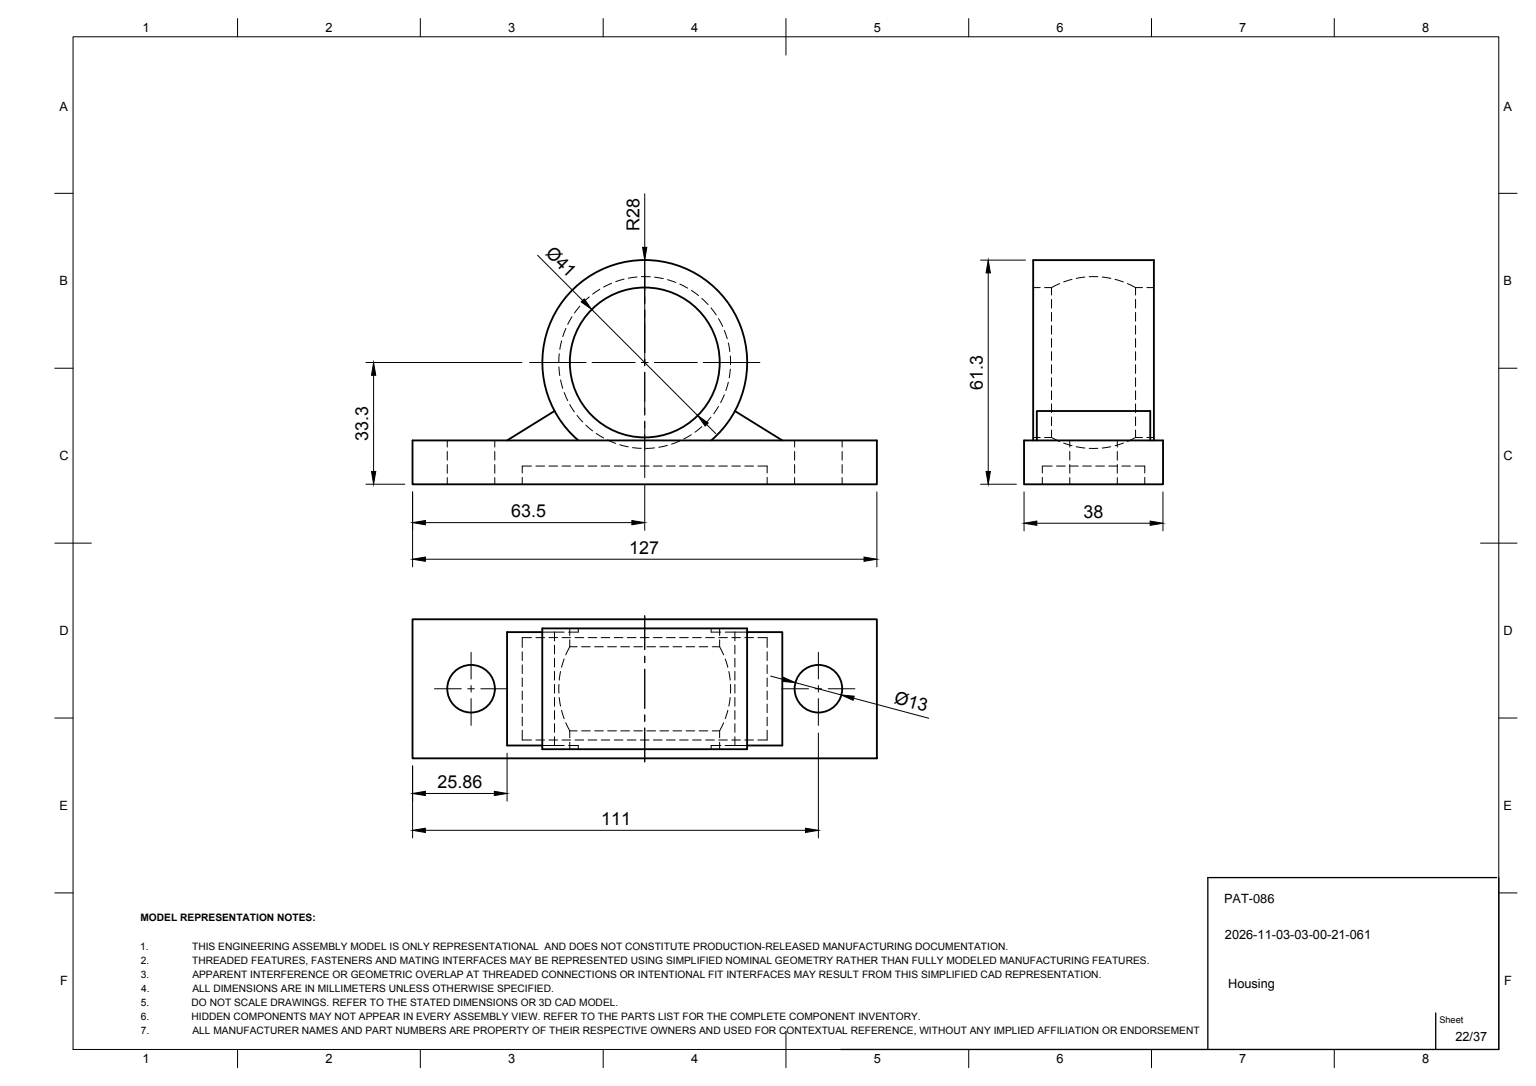
ISO-10303-21;
HEADER;
/* Generated by software containing ST-Developer
 * from STEP Tools, Inc. (www.steptools.com) 
 */

FILE_DESCRIPTION(
/* description */ ('Ratchet and pawl hand winch drum'),
/* implementation_level */ '2;1');

FILE_NAME(
/* name */ 'Housing.step',
/* time_stamp */ '2026-10-27T12:42:58-07:00',
/* author */ (''),
/* organization */ (''),
/* preprocessor_version */ 'ST-DEVELOPER v20.2',
/* originating_system */ 'Autodesk Translation Framework v15.17.0.0',
/* authorisation */ '');

FILE_SCHEMA (('AUTOMOTIVE_DESIGN { 1 0 10303 214 3 1 1 }'));
ENDSEC;

DATA;
#10=MECHANICAL_DESIGN_GEOMETRIC_PRESENTATION_REPRESENTATION('',(#404),#11801);
#319=SPHERICAL_SURFACE('',#6928,2.35);
#336=SHAPE_REPRESENTATION_RELATIONSHIP('SRR','None',#11963,#370);
#370=ADVANCED_BREP_SHAPE_REPRESENTATION('',(#439),#11780);
#404=STYLED_ITEM('',(#12192),#439);
#439=MANIFOLD_SOLID_BREP('Body1',#6281);
#531=FACE_BOUND('',#1400,.T.);
#532=FACE_BOUND('',#1401,.T.);
#533=FACE_BOUND('',#1409,.T.);
#534=FACE_BOUND('',#1410,.T.);
#535=FACE_BOUND('',#1411,.T.);
#536=FACE_BOUND('',#1414,.T.);
#537=FACE_BOUND('',#1416,.T.);
#538=FACE_BOUND('',#1429,.T.);
#539=FACE_BOUND('',#1430,.T.);
#540=FACE_BOUND('',#1431,.T.);
#678=PLANE('',#6930);
#679=PLANE('',#6932);
#680=PLANE('',#6934);
#681=PLANE('',#6936);
#682=PLANE('',#6937);
#683=PLANE('',#6939);
#684=PLANE('',#6940);
#685=PLANE('',#6946);
#686=PLANE('',#6947);
#687=PLANE('',#6948);
#688=PLANE('',#6949);
#689=PLANE('',#6950);
#690=PLANE('',#6951);
#691=PLANE('',#6952);
#692=PLANE('',#6957);
#693=PLANE('',#6958);
#694=PLANE('',#6959);
#695=PLANE('',#6960);
#696=PLANE('',#6961);
#966=FACE_OUTER_BOUND('',#1397,.T.);
#967=FACE_OUTER_BOUND('',#1398,.T.);
#968=FACE_OUTER_BOUND('',#1399,.T.);
#969=FACE_OUTER_BOUND('',#1402,.T.);
#970=FACE_OUTER_BOUND('',#1403,.T.);
#971=FACE_OUTER_BOUND('',#1404,.T.);
#972=FACE_OUTER_BOUND('',#1405,.T.);
#973=FACE_OUTER_BOUND('',#1406,.T.);
#974=FACE_OUTER_BOUND('',#1407,.T.);
#975=FACE_OUTER_BOUND('',#1408,.T.);
#976=FACE_OUTER_BOUND('',#1412,.T.);
#977=FACE_OUTER_BOUND('',#1413,.T.);
#978=FACE_OUTER_BOUND('',#1415,.T.);
#979=FACE_OUTER_BOUND('',#1417,.T.);
#980=FACE_OUTER_BOUND('',#1418,.T.);
#981=FACE_OUTER_BOUND('',#1419,.T.);
#982=FACE_OUTER_BOUND('',#1420,.T.);
#983=FACE_OUTER_BOUND('',#1421,.T.);
#984=FACE_OUTER_BOUND('',#1422,.T.);
#985=FACE_OUTER_BOUND('',#1423,.T.);
#986=FACE_OUTER_BOUND('',#1424,.T.);
#987=FACE_OUTER_BOUND('',#1425,.T.);
#988=FACE_OUTER_BOUND('',#1426,.T.);
#989=FACE_OUTER_BOUND('',#1427,.T.);
#990=FACE_OUTER_BOUND('',#1428,.T.);
#1397=EDGE_LOOP('',(#4757,#4758,#4759,#4760));
#1398=EDGE_LOOP('',(#4761,#4762,#4763,#4764));
#1399=EDGE_LOOP('',(#4765,#4766));
#1400=EDGE_LOOP('',(#4767));
#1401=EDGE_LOOP('',(#4768));
#1402=EDGE_LOOP('',(#4769,#4770,#4771));
#1403=EDGE_LOOP('',(#4772,#4773,#4774));
#1404=EDGE_LOOP('',(#4775,#4776,#4777));
#1405=EDGE_LOOP('',(#4778,#4779,#4780,#4781));
#1406=EDGE_LOOP('',(#4782,#4783,#4784));
#1407=EDGE_LOOP('',(#4785,#4786,#4787,#4788));
#1408=EDGE_LOOP('',(#4789,#4790,#4791,#4792));
#1409=EDGE_LOOP('',(#4793));
#1410=EDGE_LOOP('',(#4794));
#1411=EDGE_LOOP('',(#4795,#4796,#4797,#4798,#4799,#4800,#4801,#4802,#4803,
#4804,#4805,#4806));
#1412=EDGE_LOOP('',(#4807,#4808,#4809,#4810,#4811,#4812,#4813,#4814,#4815,
#4816,#4817,#4818));
#1413=EDGE_LOOP('',(#4819,#4820));
#1414=EDGE_LOOP('',(#4821));
#1415=EDGE_LOOP('',(#4822,#4823));
#1416=EDGE_LOOP('',(#4824));
#1417=EDGE_LOOP('',(#4825,#4826,#4827,#4828));
#1418=EDGE_LOOP('',(#4829,#4830,#4831,#4832));
#1419=EDGE_LOOP('',(#4833,#4834,#4835,#4836));
#1420=EDGE_LOOP('',(#4837,#4838,#4839,#4840));
#1421=EDGE_LOOP('',(#4841,#4842,#4843,#4844));
#1422=EDGE_LOOP('',(#4845,#4846,#4847,#4848));
#1423=EDGE_LOOP('',(#4849,#4850,#4851,#4852));
#1424=EDGE_LOOP('',(#4853,#4854,#4855,#4856));
#1425=EDGE_LOOP('',(#4857,#4858,#4859,#4860));
#1426=EDGE_LOOP('',(#4861,#4862,#4863,#4864));
#1427=EDGE_LOOP('',(#4865,#4866,#4867,#4868));
#1428=EDGE_LOOP('',(#4869,#4870,#4871,#4872));
#1429=EDGE_LOOP('',(#4873,#4874,#4875,#4876));
#1430=EDGE_LOOP('',(#4877));
#1431=EDGE_LOOP('',(#4878));
#1854=LINE('',#9801,#2365);
#1855=LINE('',#9807,#2366);
#1856=LINE('',#9816,#2367);
#1857=LINE('',#9818,#2368);
#1858=LINE('',#9823,#2369);
#1859=LINE('',#9826,#2370);
#1860=LINE('',#9830,#2371);
#1861=LINE('',#9833,#2372);
#1862=LINE('',#9835,#2373);
#1863=LINE('',#9836,#2374);
#1864=LINE('',#9840,#2375);
#1865=LINE('',#9842,#2376);
#1866=LINE('',#9845,#2377);
#1867=LINE('',#9846,#2378);
#1868=LINE('',#9850,#2379);
#1869=LINE('',#9852,#2380);
#1870=LINE('',#9854,#2381);
#1871=LINE('',#9855,#2382);
#1872=LINE('',#9861,#2383);
#1873=LINE('',#9863,#2384);
#1874=LINE('',#9864,#2385);
#1875=LINE('',#9866,#2386);
#1876=LINE('',#9868,#2387);
#1877=LINE('',#9869,#2388);
#1878=LINE('',#9878,#2389);
#1879=LINE('',#9880,#2390);
#1880=LINE('',#9882,#2391);
#1881=LINE('',#9883,#2392);
#1882=LINE('',#9886,#2393);
#1883=LINE('',#9888,#2394);
#1884=LINE('',#9889,#2395);
#1885=LINE('',#9892,#2396);
#1886=LINE('',#9894,#2397);
#1887=LINE('',#9895,#2398);
#1888=LINE('',#9897,#2399);
#1889=LINE('',#9898,#2400);
#1890=LINE('',#9903,#2401);
#1891=LINE('',#9907,#2402);
#1892=LINE('',#9911,#2403);
#1893=LINE('',#9912,#2404);
#1894=LINE('',#9913,#2405);
#1895=LINE('',#9916,#2406);
#1896=LINE('',#9917,#2407);
#1897=LINE('',#9920,#2408);
#1898=LINE('',#9921,#2409);
#1899=LINE('',#9923,#2410);
#2365=VECTOR('',#8005,2.05);
#2366=VECTOR('',#8012,2.05);
#2367=VECTOR('',#8021,1.);
#2368=VECTOR('',#8022,1.);
#2369=VECTOR('',#8027,1.);
#2370=VECTOR('',#8030,1.);
#2371=VECTOR('',#8033,1.);
#2372=VECTOR('',#8036,1.);
#2373=VECTOR('',#8039,1.);
#2374=VECTOR('',#8040,1.);
#2375=VECTOR('',#8043,1.);
#2376=VECTOR('',#8044,1.);
#2377=VECTOR('',#8049,1.);
#2378=VECTOR('',#8050,1.);
#2379=VECTOR('',#8053,1.);
#2380=VECTOR('',#8054,1.);
#2381=VECTOR('',#8055,1.);
#2382=VECTOR('',#8056,1.);
#2383=VECTOR('',#8061,1.);
#2384=VECTOR('',#8062,1.);
#2385=VECTOR('',#8063,1.);
#2386=VECTOR('',#8064,1.);
#2387=VECTOR('',#8065,1.);
#2388=VECTOR('',#8066,1.);
#2389=VECTOR('',#8079,1.);
#2390=VECTOR('',#8080,1.);
#2391=VECTOR('',#8081,1.);
#2392=VECTOR('',#8082,1.);
#2393=VECTOR('',#8085,1.);
#2394=VECTOR('',#8086,1.);
#2395=VECTOR('',#8087,1.);
#2396=VECTOR('',#8090,1.);
#2397=VECTOR('',#8091,1.);
#2398=VECTOR('',#8092,1.);
#2399=VECTOR('',#8095,1.);
#2400=VECTOR('',#8096,1.);
#2401=VECTOR('',#8103,0.65);
#2402=VECTOR('',#8108,0.65);
#2403=VECTOR('',#8111,1.);
#2404=VECTOR('',#8112,1.);
#2405=VECTOR('',#8113,1.);
#2406=VECTOR('',#8116,1.);
#2407=VECTOR('',#8117,1.);
#2408=VECTOR('',#8120,1.);
#2409=VECTOR('',#8121,1.);
#2410=VECTOR('',#8124,1.);
#2817=CIRCLE('',#6923,2.05);
#2818=CIRCLE('',#6924,2.05);
#2819=CIRCLE('',#6926,2.05);
#2820=CIRCLE('',#6927,2.05);
#2821=CIRCLE('',#6929,2.35);
#2822=CIRCLE('',#6931,2.8);
#2823=CIRCLE('',#6933,2.8);
#2824=CIRCLE('',#6935,2.8);
#2825=CIRCLE('',#6938,2.8);
#2826=CIRCLE('',#6941,0.65);
#2827=CIRCLE('',#6942,0.65);
#2828=CIRCLE('',#6944,2.8);
#2829=CIRCLE('',#6945,2.8);
#2830=CIRCLE('',#6954,0.65);
#2831=CIRCLE('',#6956,0.65);
#3112=VERTEX_POINT('',#9798);
#3113=VERTEX_POINT('',#9800);
#3114=VERTEX_POINT('',#9804);
#3115=VERTEX_POINT('',#9806);
#3116=VERTEX_POINT('',#9810);
#3117=VERTEX_POINT('',#9811);
#3118=VERTEX_POINT('',#9814);
#3119=VERTEX_POINT('',#9815);
#3120=VERTEX_POINT('',#9817);
#3121=VERTEX_POINT('',#9821);
#3122=VERTEX_POINT('',#9822);
#3123=VERTEX_POINT('',#9824);
#3124=VERTEX_POINT('',#9828);
#3125=VERTEX_POINT('',#9829);
#3126=VERTEX_POINT('',#9831);
#3127=VERTEX_POINT('',#9838);
#3128=VERTEX_POINT('',#9839);
#3129=VERTEX_POINT('',#9841);
#3130=VERTEX_POINT('',#9848);
#3131=VERTEX_POINT('',#9849);
#3132=VERTEX_POINT('',#9851);
#3133=VERTEX_POINT('',#9853);
#3134=VERTEX_POINT('',#9856);
#3135=VERTEX_POINT('',#9858);
#3136=VERTEX_POINT('',#9860);
#3137=VERTEX_POINT('',#9862);
#3138=VERTEX_POINT('',#9865);
#3139=VERTEX_POINT('',#9867);
#3140=VERTEX_POINT('',#9876);
#3141=VERTEX_POINT('',#9877);
#3142=VERTEX_POINT('',#9879);
#3143=VERTEX_POINT('',#9881);
#3144=VERTEX_POINT('',#9885);
#3145=VERTEX_POINT('',#9887);
#3146=VERTEX_POINT('',#9891);
#3147=VERTEX_POINT('',#9893);
#3148=VERTEX_POINT('',#9901);
#3149=VERTEX_POINT('',#9905);
#3150=VERTEX_POINT('',#9909);
#3151=VERTEX_POINT('',#9910);
#3152=VERTEX_POINT('',#9915);
#3153=VERTEX_POINT('',#9919);
#3722=EDGE_CURVE('',#3112,#3112,#2817,.T.);
#3723=EDGE_CURVE('',#3112,#3113,#1854,.T.);
#3724=EDGE_CURVE('',#3113,#3113,#2818,.T.);
#3725=EDGE_CURVE('',#3114,#3114,#2819,.T.);
#3726=EDGE_CURVE('',#3114,#3115,#1855,.T.);
#3727=EDGE_CURVE('',#3115,#3115,#2820,.T.);
#3728=EDGE_CURVE('',#3116,#3117,#2821,.T.);
#3729=EDGE_CURVE('',#3118,#3119,#1856,.T.);
#3730=EDGE_CURVE('',#3118,#3120,#1857,.T.);
#3731=EDGE_CURVE('',#3119,#3120,#2822,.T.);
#3732=EDGE_CURVE('',#3121,#3122,#1858,.T.);
#3733=EDGE_CURVE('',#3123,#3121,#2823,.T.);
#3734=EDGE_CURVE('',#3123,#3122,#1859,.T.);
#3735=EDGE_CURVE('',#3124,#3125,#1860,.T.);
#3736=EDGE_CURVE('',#3126,#3124,#2824,.T.);
#3737=EDGE_CURVE('',#3126,#3125,#1861,.T.);
#3738=EDGE_CURVE('',#3125,#3118,#1862,.T.);
#3739=EDGE_CURVE('',#3120,#3126,#1863,.T.);
#3740=EDGE_CURVE('',#3127,#3128,#1864,.T.);
#3741=EDGE_CURVE('',#3127,#3129,#1865,.T.);
#3742=EDGE_CURVE('',#3128,#3129,#2825,.T.);
#3743=EDGE_CURVE('',#3122,#3127,#1866,.T.);
#3744=EDGE_CURVE('',#3129,#3123,#1867,.T.);
#3745=EDGE_CURVE('',#3130,#3131,#1868,.T.);
#3746=EDGE_CURVE('',#3131,#3132,#1869,.T.);
#3747=EDGE_CURVE('',#3132,#3133,#1870,.T.);
#3748=EDGE_CURVE('',#3133,#3130,#1871,.T.);
#3749=EDGE_CURVE('',#3134,#3134,#2826,.T.);
#3750=EDGE_CURVE('',#3135,#3135,#2827,.T.);
#3751=EDGE_CURVE('',#3128,#3136,#1872,.T.);
#3752=EDGE_CURVE('',#3136,#3137,#1873,.T.);
#3753=EDGE_CURVE('',#3137,#3124,#1874,.T.);
#3754=EDGE_CURVE('',#3119,#3138,#1875,.T.);
#3755=EDGE_CURVE('',#3138,#3139,#1876,.T.);
#3756=EDGE_CURVE('',#3139,#3121,#1877,.T.);
#3757=EDGE_CURVE('',#3138,#3139,#2828,.T.);
#3758=EDGE_CURVE('',#3136,#3137,#2829,.T.);
#3759=EDGE_CURVE('',#3140,#3141,#1878,.T.);
#3760=EDGE_CURVE('',#3140,#3142,#1879,.T.);
#3761=EDGE_CURVE('',#3142,#3143,#1880,.T.);
#3762=EDGE_CURVE('',#3141,#3143,#1881,.T.);
#3763=EDGE_CURVE('',#3144,#3140,#1882,.T.);
#3764=EDGE_CURVE('',#3144,#3145,#1883,.T.);
#3765=EDGE_CURVE('',#3145,#3142,#1884,.T.);
#3766=EDGE_CURVE('',#3146,#3144,#1885,.T.);
#3767=EDGE_CURVE('',#3146,#3147,#1886,.T.);
#3768=EDGE_CURVE('',#3147,#3145,#1887,.T.);
#3769=EDGE_CURVE('',#3141,#3146,#1888,.T.);
#3770=EDGE_CURVE('',#3143,#3147,#1889,.T.);
#3771=EDGE_CURVE('',#3148,#3148,#2830,.T.);
#3772=EDGE_CURVE('',#3148,#3135,#1890,.T.);
#3773=EDGE_CURVE('',#3149,#3149,#2831,.T.);
#3774=EDGE_CURVE('',#3149,#3134,#1891,.T.);
#3775=EDGE_CURVE('',#3150,#3151,#1892,.T.);
#3776=EDGE_CURVE('',#3151,#3130,#1893,.T.);
#3777=EDGE_CURVE('',#3150,#3133,#1894,.T.);
#3778=EDGE_CURVE('',#3152,#3150,#1895,.T.);
#3779=EDGE_CURVE('',#3152,#3132,#1896,.T.);
#3780=EDGE_CURVE('',#3153,#3152,#1897,.T.);
#3781=EDGE_CURVE('',#3153,#3131,#1898,.T.);
#3782=EDGE_CURVE('',#3151,#3153,#1899,.T.);
#4757=ORIENTED_EDGE('',*,*,#3722,.F.);
#4758=ORIENTED_EDGE('',*,*,#3723,.T.);
#4759=ORIENTED_EDGE('',*,*,#3724,.F.);
#4760=ORIENTED_EDGE('',*,*,#3723,.F.);
#4761=ORIENTED_EDGE('',*,*,#3725,.F.);
#4762=ORIENTED_EDGE('',*,*,#3726,.T.);
#4763=ORIENTED_EDGE('',*,*,#3727,.F.);
#4764=ORIENTED_EDGE('',*,*,#3726,.F.);
#4765=ORIENTED_EDGE('',*,*,#3728,.T.);
#4766=ORIENTED_EDGE('',*,*,#3728,.F.);
#4767=ORIENTED_EDGE('',*,*,#3725,.T.);
#4768=ORIENTED_EDGE('',*,*,#3724,.T.);
#4769=ORIENTED_EDGE('',*,*,#3729,.F.);
#4770=ORIENTED_EDGE('',*,*,#3730,.T.);
#4771=ORIENTED_EDGE('',*,*,#3731,.F.);
#4772=ORIENTED_EDGE('',*,*,#3732,.F.);
#4773=ORIENTED_EDGE('',*,*,#3733,.F.);
#4774=ORIENTED_EDGE('',*,*,#3734,.T.);
#4775=ORIENTED_EDGE('',*,*,#3735,.F.);
#4776=ORIENTED_EDGE('',*,*,#3736,.F.);
#4777=ORIENTED_EDGE('',*,*,#3737,.T.);
#4778=ORIENTED_EDGE('',*,*,#3738,.F.);
#4779=ORIENTED_EDGE('',*,*,#3737,.F.);
#4780=ORIENTED_EDGE('',*,*,#3739,.F.);
#4781=ORIENTED_EDGE('',*,*,#3730,.F.);
#4782=ORIENTED_EDGE('',*,*,#3740,.F.);
#4783=ORIENTED_EDGE('',*,*,#3741,.T.);
#4784=ORIENTED_EDGE('',*,*,#3742,.F.);
#4785=ORIENTED_EDGE('',*,*,#3743,.F.);
#4786=ORIENTED_EDGE('',*,*,#3734,.F.);
#4787=ORIENTED_EDGE('',*,*,#3744,.F.);
#4788=ORIENTED_EDGE('',*,*,#3741,.F.);
#4789=ORIENTED_EDGE('',*,*,#3745,.T.);
#4790=ORIENTED_EDGE('',*,*,#3746,.T.);
#4791=ORIENTED_EDGE('',*,*,#3747,.T.);
#4792=ORIENTED_EDGE('',*,*,#3748,.T.);
#4793=ORIENTED_EDGE('',*,*,#3749,.T.);
#4794=ORIENTED_EDGE('',*,*,#3750,.T.);
#4795=ORIENTED_EDGE('',*,*,#3732,.T.);
#4796=ORIENTED_EDGE('',*,*,#3743,.T.);
#4797=ORIENTED_EDGE('',*,*,#3740,.T.);
#4798=ORIENTED_EDGE('',*,*,#3751,.T.);
#4799=ORIENTED_EDGE('',*,*,#3752,.T.);
#4800=ORIENTED_EDGE('',*,*,#3753,.T.);
#4801=ORIENTED_EDGE('',*,*,#3735,.T.);
#4802=ORIENTED_EDGE('',*,*,#3738,.T.);
#4803=ORIENTED_EDGE('',*,*,#3729,.T.);
#4804=ORIENTED_EDGE('',*,*,#3754,.T.);
#4805=ORIENTED_EDGE('',*,*,#3755,.T.);
#4806=ORIENTED_EDGE('',*,*,#3756,.T.);
#4807=ORIENTED_EDGE('',*,*,#3733,.T.);
#4808=ORIENTED_EDGE('',*,*,#3756,.F.);
#4809=ORIENTED_EDGE('',*,*,#3757,.F.);
#4810=ORIENTED_EDGE('',*,*,#3754,.F.);
#4811=ORIENTED_EDGE('',*,*,#3731,.T.);
#4812=ORIENTED_EDGE('',*,*,#3739,.T.);
#4813=ORIENTED_EDGE('',*,*,#3736,.T.);
#4814=ORIENTED_EDGE('',*,*,#3753,.F.);
#4815=ORIENTED_EDGE('',*,*,#3758,.F.);
#4816=ORIENTED_EDGE('',*,*,#3751,.F.);
#4817=ORIENTED_EDGE('',*,*,#3742,.T.);
#4818=ORIENTED_EDGE('',*,*,#3744,.T.);
#4819=ORIENTED_EDGE('',*,*,#3752,.F.);
#4820=ORIENTED_EDGE('',*,*,#3758,.T.);
#4821=ORIENTED_EDGE('',*,*,#3722,.T.);
#4822=ORIENTED_EDGE('',*,*,#3755,.F.);
#4823=ORIENTED_EDGE('',*,*,#3757,.T.);
#4824=ORIENTED_EDGE('',*,*,#3727,.T.);
#4825=ORIENTED_EDGE('',*,*,#3759,.F.);
#4826=ORIENTED_EDGE('',*,*,#3760,.T.);
#4827=ORIENTED_EDGE('',*,*,#3761,.T.);
#4828=ORIENTED_EDGE('',*,*,#3762,.F.);
#4829=ORIENTED_EDGE('',*,*,#3763,.F.);
#4830=ORIENTED_EDGE('',*,*,#3764,.T.);
#4831=ORIENTED_EDGE('',*,*,#3765,.T.);
#4832=ORIENTED_EDGE('',*,*,#3760,.F.);
#4833=ORIENTED_EDGE('',*,*,#3766,.F.);
#4834=ORIENTED_EDGE('',*,*,#3767,.T.);
#4835=ORIENTED_EDGE('',*,*,#3768,.T.);
#4836=ORIENTED_EDGE('',*,*,#3764,.F.);
#4837=ORIENTED_EDGE('',*,*,#3769,.F.);
#4838=ORIENTED_EDGE('',*,*,#3762,.T.);
#4839=ORIENTED_EDGE('',*,*,#3770,.T.);
#4840=ORIENTED_EDGE('',*,*,#3767,.F.);
#4841=ORIENTED_EDGE('',*,*,#3770,.F.);
#4842=ORIENTED_EDGE('',*,*,#3761,.F.);
#4843=ORIENTED_EDGE('',*,*,#3765,.F.);
#4844=ORIENTED_EDGE('',*,*,#3768,.F.);
#4845=ORIENTED_EDGE('',*,*,#3771,.F.);
#4846=ORIENTED_EDGE('',*,*,#3772,.T.);
#4847=ORIENTED_EDGE('',*,*,#3750,.F.);
#4848=ORIENTED_EDGE('',*,*,#3772,.F.);
#4849=ORIENTED_EDGE('',*,*,#3773,.F.);
#4850=ORIENTED_EDGE('',*,*,#3774,.T.);
#4851=ORIENTED_EDGE('',*,*,#3749,.F.);
#4852=ORIENTED_EDGE('',*,*,#3774,.F.);
#4853=ORIENTED_EDGE('',*,*,#3775,.T.);
#4854=ORIENTED_EDGE('',*,*,#3776,.T.);
#4855=ORIENTED_EDGE('',*,*,#3748,.F.);
#4856=ORIENTED_EDGE('',*,*,#3777,.F.);
#4857=ORIENTED_EDGE('',*,*,#3778,.T.);
#4858=ORIENTED_EDGE('',*,*,#3777,.T.);
#4859=ORIENTED_EDGE('',*,*,#3747,.F.);
#4860=ORIENTED_EDGE('',*,*,#3779,.F.);
#4861=ORIENTED_EDGE('',*,*,#3780,.T.);
#4862=ORIENTED_EDGE('',*,*,#3779,.T.);
#4863=ORIENTED_EDGE('',*,*,#3746,.F.);
#4864=ORIENTED_EDGE('',*,*,#3781,.F.);
#4865=ORIENTED_EDGE('',*,*,#3782,.T.);
#4866=ORIENTED_EDGE('',*,*,#3781,.T.);
#4867=ORIENTED_EDGE('',*,*,#3745,.F.);
#4868=ORIENTED_EDGE('',*,*,#3776,.F.);
#4869=ORIENTED_EDGE('',*,*,#3782,.F.);
#4870=ORIENTED_EDGE('',*,*,#3775,.F.);
#4871=ORIENTED_EDGE('',*,*,#3778,.F.);
#4872=ORIENTED_EDGE('',*,*,#3780,.F.);
#4873=ORIENTED_EDGE('',*,*,#3759,.T.);
#4874=ORIENTED_EDGE('',*,*,#3769,.T.);
#4875=ORIENTED_EDGE('',*,*,#3766,.T.);
#4876=ORIENTED_EDGE('',*,*,#3763,.T.);
#4877=ORIENTED_EDGE('',*,*,#3771,.T.);
#4878=ORIENTED_EDGE('',*,*,#3773,.T.);
#5856=CYLINDRICAL_SURFACE('',#6922,2.05);
#5857=CYLINDRICAL_SURFACE('',#6925,2.05);
#5858=CYLINDRICAL_SURFACE('',#6943,2.8);
#5859=CYLINDRICAL_SURFACE('',#6953,0.65);
#5860=CYLINDRICAL_SURFACE('',#6955,0.65);
#6036=ADVANCED_FACE('',(#966),#5856,.F.);
#6037=ADVANCED_FACE('',(#967),#5857,.F.);
#6038=ADVANCED_FACE('',(#968,#531,#532),#319,.F.);
#6039=ADVANCED_FACE('',(#969),#678,.T.);
#6040=ADVANCED_FACE('',(#970),#679,.T.);
#6041=ADVANCED_FACE('',(#971),#680,.T.);
#6042=ADVANCED_FACE('',(#972),#681,.T.);
#6043=ADVANCED_FACE('',(#973),#682,.T.);
#6044=ADVANCED_FACE('',(#974),#683,.T.);
#6045=ADVANCED_FACE('',(#975,#533,#534,#535),#684,.T.);
#6046=ADVANCED_FACE('',(#976),#5858,.T.);
#6047=ADVANCED_FACE('',(#977,#536),#685,.F.);
#6048=ADVANCED_FACE('',(#978,#537),#686,.T.);
#6049=ADVANCED_FACE('',(#979),#687,.F.);
#6050=ADVANCED_FACE('',(#980),#688,.F.);
#6051=ADVANCED_FACE('',(#981),#689,.F.);
#6052=ADVANCED_FACE('',(#982),#690,.F.);
#6053=ADVANCED_FACE('',(#983),#691,.F.);
#6054=ADVANCED_FACE('',(#984),#5859,.F.);
#6055=ADVANCED_FACE('',(#985),#5860,.F.);
#6056=ADVANCED_FACE('',(#986),#692,.T.);
#6057=ADVANCED_FACE('',(#987),#693,.T.);
#6058=ADVANCED_FACE('',(#988),#694,.T.);
#6059=ADVANCED_FACE('',(#989),#695,.T.);
#6060=ADVANCED_FACE('',(#990,#538,#539,#540),#696,.F.);
#6281=CLOSED_SHELL('',(#6036,#6037,#6038,#6039,#6040,#6041,#6042,#6043,
#6044,#6045,#6046,#6047,#6048,#6049,#6050,#6051,#6052,#6053,#6054,#6055,
#6056,#6057,#6058,#6059,#6060));
#6921=AXIS2_PLACEMENT_3D('',#9796,#7999,#8000);
#6922=AXIS2_PLACEMENT_3D('',#9797,#8001,#8002);
#6923=AXIS2_PLACEMENT_3D('',#9799,#8003,#8004);
#6924=AXIS2_PLACEMENT_3D('',#9802,#8006,#8007);
#6925=AXIS2_PLACEMENT_3D('',#9803,#8008,#8009);
#6926=AXIS2_PLACEMENT_3D('',#9805,#8010,#8011);
#6927=AXIS2_PLACEMENT_3D('',#9808,#8013,#8014);
#6928=AXIS2_PLACEMENT_3D('',#9809,#8015,#8016);
#6929=AXIS2_PLACEMENT_3D('',#9812,#8017,#8018);
#6930=AXIS2_PLACEMENT_3D('',#9813,#8019,#8020);
#6931=AXIS2_PLACEMENT_3D('',#9819,#8023,#8024);
#6932=AXIS2_PLACEMENT_3D('',#9820,#8025,#8026);
#6933=AXIS2_PLACEMENT_3D('',#9825,#8028,#8029);
#6934=AXIS2_PLACEMENT_3D('',#9827,#8031,#8032);
#6935=AXIS2_PLACEMENT_3D('',#9832,#8034,#8035);
#6936=AXIS2_PLACEMENT_3D('',#9834,#8037,#8038);
#6937=AXIS2_PLACEMENT_3D('',#9837,#8041,#8042);
#6938=AXIS2_PLACEMENT_3D('',#9843,#8045,#8046);
#6939=AXIS2_PLACEMENT_3D('',#9844,#8047,#8048);
#6940=AXIS2_PLACEMENT_3D('',#9847,#8051,#8052);
#6941=AXIS2_PLACEMENT_3D('',#9857,#8057,#8058);
#6942=AXIS2_PLACEMENT_3D('',#9859,#8059,#8060);
#6943=AXIS2_PLACEMENT_3D('',#9870,#8067,#8068);
#6944=AXIS2_PLACEMENT_3D('',#9871,#8069,#8070);
#6945=AXIS2_PLACEMENT_3D('',#9872,#8071,#8072);
#6946=AXIS2_PLACEMENT_3D('',#9873,#8073,#8074);
#6947=AXIS2_PLACEMENT_3D('',#9874,#8075,#8076);
#6948=AXIS2_PLACEMENT_3D('',#9875,#8077,#8078);
#6949=AXIS2_PLACEMENT_3D('',#9884,#8083,#8084);
#6950=AXIS2_PLACEMENT_3D('',#9890,#8088,#8089);
#6951=AXIS2_PLACEMENT_3D('',#9896,#8093,#8094);
#6952=AXIS2_PLACEMENT_3D('',#9899,#8097,#8098);
#6953=AXIS2_PLACEMENT_3D('',#9900,#8099,#8100);
#6954=AXIS2_PLACEMENT_3D('',#9902,#8101,#8102);
#6955=AXIS2_PLACEMENT_3D('',#9904,#8104,#8105);
#6956=AXIS2_PLACEMENT_3D('',#9906,#8106,#8107);
#6957=AXIS2_PLACEMENT_3D('',#9908,#8109,#8110);
#6958=AXIS2_PLACEMENT_3D('',#9914,#8114,#8115);
#6959=AXIS2_PLACEMENT_3D('',#9918,#8118,#8119);
#6960=AXIS2_PLACEMENT_3D('',#9922,#8122,#8123);
#6961=AXIS2_PLACEMENT_3D('',#9924,#8125,#8126);
#7999=DIRECTION('axis',(0.,0.,1.));
#8000=DIRECTION('refdir',(1.,0.,0.));
#8001=DIRECTION('center_axis',(0.,1.,0.));
#8002=DIRECTION('ref_axis',(1.,0.,0.));
#8003=DIRECTION('center_axis',(0.,1.,0.));
#8004=DIRECTION('ref_axis',(1.,0.,0.));
#8005=DIRECTION('',(0.,1.,0.));
#8006=DIRECTION('center_axis',(0.,-1.,0.));
#8007=DIRECTION('ref_axis',(1.,0.,0.));
#8008=DIRECTION('center_axis',(0.,1.,0.));
#8009=DIRECTION('ref_axis',(1.,0.,0.));
#8010=DIRECTION('center_axis',(0.,1.,0.));
#8011=DIRECTION('ref_axis',(1.,0.,0.));
#8012=DIRECTION('',(0.,1.,0.));
#8013=DIRECTION('center_axis',(0.,-1.,0.));
#8014=DIRECTION('ref_axis',(1.,0.,0.));
#8015=DIRECTION('center_axis',(6.12323399573677E-17,0.,1.));
#8016=DIRECTION('ref_axis',(1.,0.,0.));
#8017=DIRECTION('center_axis',(-1.22464679914735E-16,1.,0.));
#8018=DIRECTION('ref_axis',(-1.,-1.22464679914735E-16,0.));
#8019=DIRECTION('center_axis',(0.,1.,0.));
#8020=DIRECTION('ref_axis',(0.,0.,1.));
#8021=DIRECTION('',(1.,0.,0.));
#8022=DIRECTION('',(0.850265146687862,0.,0.526354614616295));
#8023=DIRECTION('center_axis',(0.,1.,0.));
#8024=DIRECTION('ref_axis',(1.,0.,0.));
#8025=DIRECTION('center_axis',(0.,1.,0.));
#8026=DIRECTION('ref_axis',(0.,0.,1.));
#8027=DIRECTION('',(1.,0.,0.));
#8028=DIRECTION('center_axis',(0.,1.,0.));
#8029=DIRECTION('ref_axis',(1.,0.,0.));
#8030=DIRECTION('',(0.850265146687862,0.,-0.526354614616295));
#8031=DIRECTION('center_axis',(0.,-1.,0.));
#8032=DIRECTION('ref_axis',(0.,0.,-1.));
#8033=DIRECTION('',(-1.,0.,0.));
#8034=DIRECTION('center_axis',(0.,-1.,0.));
#8035=DIRECTION('ref_axis',(1.,0.,0.));
#8036=DIRECTION('',(-0.850265146687862,0.,-0.526354614616295));
#8037=DIRECTION('center_axis',(-0.526354614616295,0.,0.850265146687862));
#8038=DIRECTION('ref_axis',(0.850265146687862,0.,0.526354614616295));
#8039=DIRECTION('',(0.,1.,0.));
#8040=DIRECTION('',(0.,-1.,0.));
#8041=DIRECTION('center_axis',(0.,-1.,0.));
#8042=DIRECTION('ref_axis',(0.,0.,-1.));
#8043=DIRECTION('',(-1.,0.,0.));
#8044=DIRECTION('',(-0.850265146687862,0.,0.526354614616295));
#8045=DIRECTION('center_axis',(0.,-1.,0.));
#8046=DIRECTION('ref_axis',(1.,0.,0.));
#8047=DIRECTION('center_axis',(0.526354614616295,0.,0.850265146687862));
#8048=DIRECTION('ref_axis',(0.850265146687862,0.,-0.526354614616295));
#8049=DIRECTION('',(0.,-1.,0.));
#8050=DIRECTION('',(0.,1.,0.));
#8051=DIRECTION('center_axis',(0.,0.,1.));
#8052=DIRECTION('ref_axis',(1.,0.,0.));
#8053=DIRECTION('',(0.,-1.,0.));
#8054=DIRECTION('',(1.,0.,0.));
#8055=DIRECTION('',(0.,1.,0.));
#8056=DIRECTION('',(-1.,0.,0.));
#8057=DIRECTION('center_axis',(0.,0.,-1.));
#8058=DIRECTION('ref_axis',(1.,0.,0.));
#8059=DIRECTION('center_axis',(0.,0.,-1.));
#8060=DIRECTION('ref_axis',(1.,0.,0.));
#8061=DIRECTION('',(0.,-1.,0.));
#8062=DIRECTION('',(-1.,0.,0.));
#8063=DIRECTION('',(0.,1.,0.));
#8064=DIRECTION('',(0.,1.,0.));
#8065=DIRECTION('',(1.,0.,0.));
#8066=DIRECTION('',(0.,-1.,0.));
#8067=DIRECTION('center_axis',(0.,1.,0.));
#8068=DIRECTION('ref_axis',(6.12323399573677E-17,0.,1.));
#8069=DIRECTION('center_axis',(0.,1.,0.));
#8070=DIRECTION('ref_axis',(1.,0.,0.));
#8071=DIRECTION('center_axis',(0.,-1.,0.));
#8072=DIRECTION('ref_axis',(1.,0.,0.));
#8073=DIRECTION('center_axis',(0.,1.,0.));
#8074=DIRECTION('ref_axis',(1.,0.,0.));
#8075=DIRECTION('center_axis',(0.,1.,0.));
#8076=DIRECTION('ref_axis',(1.,0.,0.));
#8077=DIRECTION('center_axis',(0.,1.,0.));
#8078=DIRECTION('ref_axis',(-1.,0.,0.));
#8079=DIRECTION('',(-1.,0.,0.));
#8080=DIRECTION('',(0.,0.,1.));
#8081=DIRECTION('',(-1.,0.,0.));
#8082=DIRECTION('',(0.,0.,1.));
#8083=DIRECTION('center_axis',(1.,0.,0.));
#8084=DIRECTION('ref_axis',(0.,1.,0.));
#8085=DIRECTION('',(0.,1.,0.));
#8086=DIRECTION('',(0.,0.,1.));
#8087=DIRECTION('',(0.,1.,0.));
#8088=DIRECTION('center_axis',(0.,-1.,0.));
#8089=DIRECTION('ref_axis',(1.,0.,0.));
#8090=DIRECTION('',(1.,0.,0.));
#8091=DIRECTION('',(0.,0.,1.));
#8092=DIRECTION('',(1.,0.,0.));
#8093=DIRECTION('center_axis',(-1.,0.,0.));
#8094=DIRECTION('ref_axis',(0.,-1.,0.));
#8095=DIRECTION('',(0.,-1.,0.));
#8096=DIRECTION('',(0.,-1.,0.));
#8097=DIRECTION('center_axis',(0.,0.,1.));
#8098=DIRECTION('ref_axis',(1.,0.,0.));
#8099=DIRECTION('center_axis',(0.,0.,1.));
#8100=DIRECTION('ref_axis',(1.,0.,0.));
#8101=DIRECTION('center_axis',(0.,0.,1.));
#8102=DIRECTION('ref_axis',(1.,0.,0.));
#8103=DIRECTION('',(0.,0.,1.));
#8104=DIRECTION('center_axis',(0.,0.,1.));
#8105=DIRECTION('ref_axis',(1.,0.,0.));
#8106=DIRECTION('center_axis',(0.,0.,1.));
#8107=DIRECTION('ref_axis',(1.,0.,0.));
#8108=DIRECTION('',(0.,0.,1.));
#8109=DIRECTION('center_axis',(0.,1.,0.));
#8110=DIRECTION('ref_axis',(-1.,0.,0.));
#8111=DIRECTION('',(-1.,0.,0.));
#8112=DIRECTION('',(0.,0.,1.));
#8113=DIRECTION('',(0.,0.,1.));
#8114=DIRECTION('center_axis',(1.,0.,0.));
#8115=DIRECTION('ref_axis',(0.,1.,0.));
#8116=DIRECTION('',(0.,1.,0.));
#8117=DIRECTION('',(0.,0.,1.));
#8118=DIRECTION('center_axis',(0.,-1.,0.));
#8119=DIRECTION('ref_axis',(1.,0.,0.));
#8120=DIRECTION('',(1.,0.,0.));
#8121=DIRECTION('',(0.,0.,1.));
#8122=DIRECTION('center_axis',(-1.,0.,0.));
#8123=DIRECTION('ref_axis',(0.,-1.,0.));
#8124=DIRECTION('',(0.,-1.,0.));
#8125=DIRECTION('center_axis',(0.,0.,1.));
#8126=DIRECTION('ref_axis',(1.,0.,0.));
#9796=CARTESIAN_POINT('',(0.,0.,0.));
#9797=CARTESIAN_POINT('Origin',(0.,0.,0.));
#9798=CARTESIAN_POINT('',(-2.05,-1.65,2.51052593825207E-16));
#9799=CARTESIAN_POINT('Origin',(0.,-1.65,0.));
#9800=CARTESIAN_POINT('',(-2.05,-1.14891252930761,-2.51052593825207E-16));
#9801=CARTESIAN_POINT('',(-2.05,0.,2.51052593825207E-16));
#9802=CARTESIAN_POINT('Origin',(0.,-1.14891252930761,0.));
#9803=CARTESIAN_POINT('Origin',(0.,0.,0.));
#9804=CARTESIAN_POINT('',(-2.05,1.14891252930761,2.51052593825207E-16));
#9805=CARTESIAN_POINT('Origin',(0.,1.14891252930761,0.));
#9806=CARTESIAN_POINT('',(-2.05,1.65,-2.51052593825207E-16));
#9807=CARTESIAN_POINT('',(-2.05,0.,2.51052593825207E-16));
#9808=CARTESIAN_POINT('Origin',(0.,1.65,0.));
#9809=CARTESIAN_POINT('Origin',(0.,0.,0.));
#9810=CARTESIAN_POINT('',(-1.43895998899814E-16,-1.76221774462768E-32,-2.35));
#9811=CARTESIAN_POINT('',(-1.43895998899814E-16,-1.76221774462768E-32,2.35));
#9812=CARTESIAN_POINT('Origin',(0.,0.,0.));
#9813=CARTESIAN_POINT('Origin',(0.,1.55,-1.49));
#9814=CARTESIAN_POINT('',(-3.76384615384615,1.55,-2.13));
#9815=CARTESIAN_POINT('',(-1.81744325908679,1.55,-2.13));
#9816=CARTESIAN_POINT('',(0.,1.55,-2.13));
#9817=CARTESIAN_POINT('',(-2.46585583768694,1.55,-1.32648218523477));
#9818=CARTESIAN_POINT('',(-1.68,1.55,-0.84));
#9819=CARTESIAN_POINT('Origin',(0.,1.55,0.));
#9820=CARTESIAN_POINT('Origin',(0.,1.55,-1.49));
#9821=CARTESIAN_POINT('',(1.81744325908679,1.55,-2.13));
#9822=CARTESIAN_POINT('',(3.76384615384615,1.55,-2.13));
#9823=CARTESIAN_POINT('',(0.,1.55,-2.13));
#9824=CARTESIAN_POINT('',(2.46585583768694,1.55,-1.32648218523477));
#9825=CARTESIAN_POINT('Origin',(0.,1.55,0.));
#9826=CARTESIAN_POINT('',(3.78,1.55,-2.14));
#9827=CARTESIAN_POINT('Origin',(0.,-1.55,-1.49));
#9828=CARTESIAN_POINT('',(-1.81744325908679,-1.55,-2.13));
#9829=CARTESIAN_POINT('',(-3.76384615384615,-1.55,-2.13));
#9830=CARTESIAN_POINT('',(0.,-1.55,-2.13));
#9831=CARTESIAN_POINT('',(-2.46585583768694,-1.55,-1.32648218523477));
#9832=CARTESIAN_POINT('Origin',(0.,-1.55,0.));
#9833=CARTESIAN_POINT('',(-1.68,-1.55,-0.84));
#9834=CARTESIAN_POINT('Origin',(-3.78,0.,-2.14));
#9835=CARTESIAN_POINT('',(-3.76384615384615,0.,-2.13));
#9836=CARTESIAN_POINT('',(-2.46585583768694,0.,-1.32648218523477));
#9837=CARTESIAN_POINT('Origin',(0.,-1.55,-1.49));
#9838=CARTESIAN_POINT('',(3.76384615384615,-1.55,-2.13));
#9839=CARTESIAN_POINT('',(1.81744325908679,-1.55,-2.13));
#9840=CARTESIAN_POINT('',(0.,-1.55,-2.13));
#9841=CARTESIAN_POINT('',(2.46585583768694,-1.55,-1.32648218523477));
#9842=CARTESIAN_POINT('',(3.78,-1.55,-2.14));
#9843=CARTESIAN_POINT('Origin',(0.,-1.55,0.));
#9844=CARTESIAN_POINT('Origin',(1.68,0.,-0.84));
#9845=CARTESIAN_POINT('',(3.76384615384615,0.,-2.13));
#9846=CARTESIAN_POINT('',(2.46585583768694,0.,-1.32648218523477));
#9847=CARTESIAN_POINT('Origin',(0.,0.,-2.13));
#9848=CARTESIAN_POINT('',(-6.35,1.9,-2.13));
#9849=CARTESIAN_POINT('',(-6.35,-1.9,-2.13));
#9850=CARTESIAN_POINT('',(-6.35,1.9,-2.13));
#9851=CARTESIAN_POINT('',(6.35,-1.9,-2.13));
#9852=CARTESIAN_POINT('',(-6.35,-1.9,-2.13));
#9853=CARTESIAN_POINT('',(6.35,1.9,-2.13));
#9854=CARTESIAN_POINT('',(6.35,-1.9,-2.13));
#9855=CARTESIAN_POINT('',(6.35,1.9,-2.13));
#9856=CARTESIAN_POINT('',(4.1,7.9602041944578E-17,-2.13));
#9857=CARTESIAN_POINT('Origin',(4.75,0.,-2.13));
#9858=CARTESIAN_POINT('',(-5.4,7.9602041944578E-17,-2.13));
#9859=CARTESIAN_POINT('Origin',(-4.75,0.,-2.13));
#9860=CARTESIAN_POINT('',(1.81744325908679,-1.65,-2.13));
#9861=CARTESIAN_POINT('',(1.81744325908679,0.,-2.13));
#9862=CARTESIAN_POINT('',(-1.81744325908679,-1.65,-2.13));
#9863=CARTESIAN_POINT('',(0.,-1.65,-2.13));
#9864=CARTESIAN_POINT('',(-1.81744325908679,0.,-2.13));
#9865=CARTESIAN_POINT('',(-1.81744325908679,1.65,-2.13));
#9866=CARTESIAN_POINT('',(-1.81744325908679,0.,-2.13));
#9867=CARTESIAN_POINT('',(1.81744325908679,1.65,-2.13));
#9868=CARTESIAN_POINT('',(0.,1.65,-2.13));
#9869=CARTESIAN_POINT('',(1.81744325908679,0.,-2.13));
#9870=CARTESIAN_POINT('Origin',(0.,0.,0.));
#9871=CARTESIAN_POINT('Origin',(0.,1.65,0.));
#9872=CARTESIAN_POINT('Origin',(0.,-1.65,0.));
#9873=CARTESIAN_POINT('Origin',(0.,-1.65,0.));
#9874=CARTESIAN_POINT('Origin',(0.,1.65,0.));
#9875=CARTESIAN_POINT('Origin',(3.35,1.4,-3.33));
#9876=CARTESIAN_POINT('',(3.35,1.4,-3.33));
#9877=CARTESIAN_POINT('',(-3.35,1.4,-3.33));
#9878=CARTESIAN_POINT('',(1.675,1.4,-3.33));
#9879=CARTESIAN_POINT('',(3.35,1.4,-2.83));
#9880=CARTESIAN_POINT('',(3.35,1.4,-3.33));
#9881=CARTESIAN_POINT('',(-3.35,1.4,-2.83));
#9882=CARTESIAN_POINT('',(3.35,1.4,-2.83));
#9883=CARTESIAN_POINT('',(-3.35,1.4,-3.33));
#9884=CARTESIAN_POINT('Origin',(3.35,-1.4,-3.33));
#9885=CARTESIAN_POINT('',(3.35,-1.4,-3.33));
#9886=CARTESIAN_POINT('',(3.35,-0.7,-3.33));
#9887=CARTESIAN_POINT('',(3.35,-1.4,-2.83));
#9888=CARTESIAN_POINT('',(3.35,-1.4,-3.33));
#9889=CARTESIAN_POINT('',(3.35,-1.4,-2.83));
#9890=CARTESIAN_POINT('Origin',(-3.35,-1.4,-3.33));
#9891=CARTESIAN_POINT('',(-3.35,-1.4,-3.33));
#9892=CARTESIAN_POINT('',(-1.675,-1.4,-3.33));
#9893=CARTESIAN_POINT('',(-3.35,-1.4,-2.83));
#9894=CARTESIAN_POINT('',(-3.35,-1.4,-3.33));
#9895=CARTESIAN_POINT('',(-3.35,-1.4,-2.83));
#9896=CARTESIAN_POINT('Origin',(-3.35,1.4,-3.33));
#9897=CARTESIAN_POINT('',(-3.35,0.7,-3.33));
#9898=CARTESIAN_POINT('',(-3.35,1.4,-2.83));
#9899=CARTESIAN_POINT('Origin',(0.,0.,-2.83));
#9900=CARTESIAN_POINT('Origin',(-4.75,0.,-3.33));
#9901=CARTESIAN_POINT('',(-5.4,-7.9602041944578E-17,-3.33));
#9902=CARTESIAN_POINT('Origin',(-4.75,0.,-3.33));
#9903=CARTESIAN_POINT('',(-5.4,-7.9602041944578E-17,-3.33));
#9904=CARTESIAN_POINT('Origin',(4.75,0.,-3.33));
#9905=CARTESIAN_POINT('',(4.1,-7.9602041944578E-17,-3.33));
#9906=CARTESIAN_POINT('Origin',(4.75,0.,-3.33));
#9907=CARTESIAN_POINT('',(4.1,-7.9602041944578E-17,-3.33));
#9908=CARTESIAN_POINT('Origin',(6.35,1.9,-3.33));
#9909=CARTESIAN_POINT('',(6.35,1.9,-3.33));
#9910=CARTESIAN_POINT('',(-6.35,1.9,-3.33));
#9911=CARTESIAN_POINT('',(6.35,1.9,-3.33));
#9912=CARTESIAN_POINT('',(-6.35,1.9,-3.33));
#9913=CARTESIAN_POINT('',(6.35,1.9,-3.33));
#9914=CARTESIAN_POINT('Origin',(6.35,-1.9,-3.33));
#9915=CARTESIAN_POINT('',(6.35,-1.9,-3.33));
#9916=CARTESIAN_POINT('',(6.35,-1.9,-3.33));
#9917=CARTESIAN_POINT('',(6.35,-1.9,-3.33));
#9918=CARTESIAN_POINT('Origin',(-6.35,-1.9,-3.33));
#9919=CARTESIAN_POINT('',(-6.35,-1.9,-3.33));
#9920=CARTESIAN_POINT('',(-6.35,-1.9,-3.33));
#9921=CARTESIAN_POINT('',(-6.35,-1.9,-3.33));
#9922=CARTESIAN_POINT('Origin',(-6.35,1.9,-3.33));
#9923=CARTESIAN_POINT('',(-6.35,1.9,-3.33));
#9924=CARTESIAN_POINT('Origin',(0.,0.,-3.33));
#11740=UNCERTAINTY_MEASURE_WITH_UNIT(LENGTH_MEASURE(0.001),#11802,
'DISTANCE_ACCURACY_VALUE',
'Maximum model space distance between geometric entities at asserted c
onnectivities');
#11761=UNCERTAINTY_MEASURE_WITH_UNIT(LENGTH_MEASURE(0.001),#11802,
'DISTANCE_ACCURACY_VALUE',
'Maximum model space distance between geometric entities at asserted c
onnectivities');
#11780=(
GEOMETRIC_REPRESENTATION_CONTEXT(3)
GLOBAL_UNCERTAINTY_ASSIGNED_CONTEXT((#11740))
GLOBAL_UNIT_ASSIGNED_CONTEXT((#11802,#11804,#11805))
REPRESENTATION_CONTEXT('','3D')
);
#11801=(
GEOMETRIC_REPRESENTATION_CONTEXT(3)
GLOBAL_UNCERTAINTY_ASSIGNED_CONTEXT((#11761))
GLOBAL_UNIT_ASSIGNED_CONTEXT((#11802,#11804,#11805))
REPRESENTATION_CONTEXT('','3D')
);
#11802=(
LENGTH_UNIT()
NAMED_UNIT(*)
SI_UNIT(.CENTI.,.METRE.)
);
#11804=(
NAMED_UNIT(*)
PLANE_ANGLE_UNIT()
SI_UNIT($,.RADIAN.)
);
#11805=(
NAMED_UNIT(*)
SI_UNIT($,.STERADIAN.)
SOLID_ANGLE_UNIT()
);
#11824=SHAPE_DEFINITION_REPRESENTATION(#11863,#11963);
#11863=PRODUCT_DEFINITION_SHAPE('',$,#12003);
#11963=SHAPE_REPRESENTATION('',(#6921),#11780);
#11984=PRODUCT_DEFINITION_CONTEXT('part definition',#12103,'design');
#12003=PRODUCT_DEFINITION('Housing','Housing',#12042,#11984);
#12042=PRODUCT_DEFINITION_FORMATION('',$,#12123);
#12103=APPLICATION_CONTEXT(
'Core Data for Automotive Mechanical Design Process');
#12104=PRODUCT_CONTEXT('part definition',#12103,'mechanical');
#12123=PRODUCT('Housing','Housing','Housing',(#12104));
#12186=COLOUR_RGB('Dark Blue',0.08,0.2,0.34);
#12187=FILL_AREA_STYLE_COLOUR('',#12186);
#12188=FILL_AREA_STYLE('',(#12187));
#12189=SURFACE_STYLE_FILL_AREA(#12188);
#12190=SURFACE_SIDE_STYLE('',(#12189));
#12191=SURFACE_STYLE_USAGE(.BOTH.,#12190);
#12192=PRESENTATION_STYLE_ASSIGNMENT((#12191));
ENDSEC;
END-ISO-10303-21;
